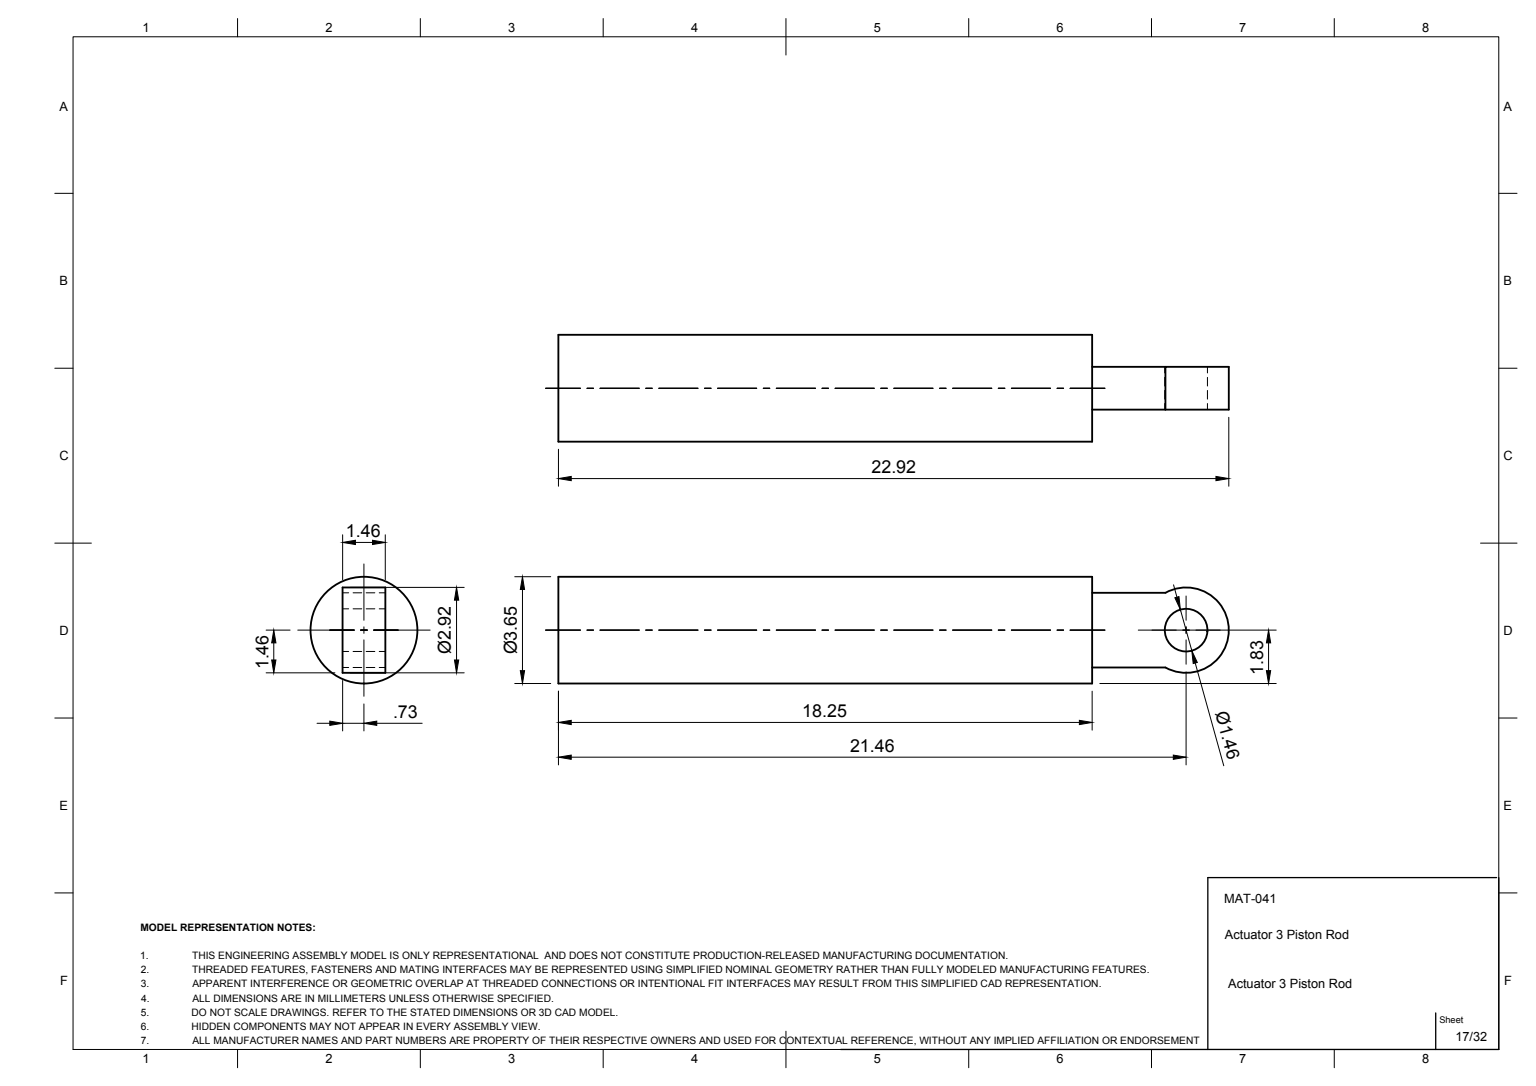
ISO-10303-21;
HEADER;
/* Generated by software containing ST-Developer
 * from STEP Tools, Inc. (www.steptools.com) 
 */

FILE_DESCRIPTION(
/* description */ ('STEP AP214'),
/* implementation_level */ '2;1');

FILE_NAME(
/* name */ 'Actuator 3 Piston Rod.step',
/* time_stamp */ '2026-11-14T21:57:47-08:00',
/* author */ (''),
/* organization */ (''),
/* preprocessor_version */ 'ST-DEVELOPER v20.2',
/* originating_system */ 'Autodesk Translation Framework v15.17.0.0',
/* authorisation */ '');

FILE_SCHEMA (('AUTOMOTIVE_DESIGN { 1 0 10303 214 3 1 1 }'));
ENDSEC;

DATA;
#10=MECHANICAL_DESIGN_GEOMETRIC_PRESENTATION_REPRESENTATION('',(#255),#13199);
#219=SHAPE_REPRESENTATION_RELATIONSHIP('SRR','None',#13289,#237);
#237=ADVANCED_BREP_SHAPE_REPRESENTATION('',(#273),#13185);
#255=STYLED_ITEM('',(#13411),#273);
#273=MANIFOLD_SOLID_BREP('Body1',#6850);
#335=FACE_BOUND('',#2475,.T.);
#336=FACE_BOUND('',#2478,.T.);
#337=FACE_BOUND('',#2481,.T.);
#505=PLANE('',#7523);
#506=PLANE('',#7524);
#507=PLANE('',#7525);
#508=PLANE('',#7526);
#509=PLANE('',#7527);
#510=PLANE('',#7528);
#898=LINE('',#11729,#1416);
#899=LINE('',#11736,#1417);
#900=LINE('',#11739,#1418);
#901=LINE('',#11744,#1419);
#902=LINE('',#11749,#1420);
#903=LINE('',#11751,#1421);
#904=LINE('',#11753,#1422);
#905=LINE('',#11754,#1423);
#906=LINE('',#11757,#1424);
#907=LINE('',#11758,#1425);
#908=LINE('',#11760,#1426);
#909=LINE('',#11762,#1427);
#1416=VECTOR('',#9029,0.730000000000001);
#1417=VECTOR('',#9036,1000.);
#1418=VECTOR('',#9039,1000.);
#1419=VECTOR('',#9044,1.825);
#1420=VECTOR('',#9049,1000.);
#1421=VECTOR('',#9050,1000.);
#1422=VECTOR('',#9051,1000.);
#1423=VECTOR('',#9052,1000.);
#1424=VECTOR('',#9057,1000.);
#1425=VECTOR('',#9058,1000.);
#1426=VECTOR('',#9061,1000.);
#1427=VECTOR('',#9064,1000.);
#1741=CYLINDRICAL_SURFACE('',#7514,0.730000000000001);
#1742=CYLINDRICAL_SURFACE('',#7517,1.46);
#1743=CYLINDRICAL_SURFACE('',#7520,1.825);
#2029=FACE_OUTER_BOUND('',#2471,.T.);
#2030=FACE_OUTER_BOUND('',#2472,.T.);
#2031=FACE_OUTER_BOUND('',#2473,.T.);
#2032=FACE_OUTER_BOUND('',#2474,.T.);
#2033=FACE_OUTER_BOUND('',#2476,.T.);
#2034=FACE_OUTER_BOUND('',#2477,.T.);
#2035=FACE_OUTER_BOUND('',#2479,.T.);
#2036=FACE_OUTER_BOUND('',#2480,.T.);
#2037=FACE_OUTER_BOUND('',#2482,.T.);
#2471=EDGE_LOOP('',(#5670,#5671,#5672,#5673));
#2472=EDGE_LOOP('',(#5674,#5675,#5676,#5677));
#2473=EDGE_LOOP('',(#5678,#5679,#5680,#5681));
#2474=EDGE_LOOP('',(#5682));
#2475=EDGE_LOOP('',(#5683,#5684,#5685,#5686));
#2476=EDGE_LOOP('',(#5687));
#2477=EDGE_LOOP('',(#5688,#5689,#5690,#5691));
#2478=EDGE_LOOP('',(#5692));
#2479=EDGE_LOOP('',(#5693,#5694,#5695,#5696));
#2480=EDGE_LOOP('',(#5697,#5698,#5699,#5700));
#2481=EDGE_LOOP('',(#5701));
#2482=EDGE_LOOP('',(#5702,#5703,#5704,#5705));
#2883=CIRCLE('',#7515,0.730000000000001);
#2884=CIRCLE('',#7516,0.730000000000001);
#2885=CIRCLE('',#7518,1.46);
#2886=CIRCLE('',#7519,1.46);
#2887=CIRCLE('',#7521,1.825);
#2888=CIRCLE('',#7522,1.825);
#3358=VERTEX_POINT('',#11726);
#3359=VERTEX_POINT('',#11728);
#3360=VERTEX_POINT('',#11732);
#3361=VERTEX_POINT('',#11733);
#3362=VERTEX_POINT('',#11735);
#3363=VERTEX_POINT('',#11737);
#3364=VERTEX_POINT('',#11741);
#3365=VERTEX_POINT('',#11743);
#3366=VERTEX_POINT('',#11747);
#3367=VERTEX_POINT('',#11748);
#3368=VERTEX_POINT('',#11750);
#3369=VERTEX_POINT('',#11752);
#4172=EDGE_CURVE('',#3358,#3358,#2883,.T.);
#4173=EDGE_CURVE('',#3358,#3359,#898,.T.);
#4174=EDGE_CURVE('',#3359,#3359,#2884,.T.);
#4175=EDGE_CURVE('',#3360,#3361,#2885,.T.);
#4176=EDGE_CURVE('',#3362,#3360,#899,.T.);
#4177=EDGE_CURVE('',#3363,#3362,#2886,.T.);
#4178=EDGE_CURVE('',#3361,#3363,#900,.T.);
#4179=EDGE_CURVE('',#3364,#3364,#2887,.T.);
#4180=EDGE_CURVE('',#3364,#3365,#901,.T.);
#4181=EDGE_CURVE('',#3365,#3365,#2888,.T.);
#4182=EDGE_CURVE('',#3366,#3367,#902,.T.);
#4183=EDGE_CURVE('',#3368,#3366,#903,.T.);
#4184=EDGE_CURVE('',#3369,#3368,#904,.T.);
#4185=EDGE_CURVE('',#3367,#3369,#905,.T.);
#4186=EDGE_CURVE('',#3363,#3366,#906,.T.);
#4187=EDGE_CURVE('',#3362,#3368,#907,.T.);
#4188=EDGE_CURVE('',#3361,#3367,#908,.T.);
#4189=EDGE_CURVE('',#3360,#3369,#909,.T.);
#5670=ORIENTED_EDGE('',*,*,#4172,.F.);
#5671=ORIENTED_EDGE('',*,*,#4173,.T.);
#5672=ORIENTED_EDGE('',*,*,#4174,.T.);
#5673=ORIENTED_EDGE('',*,*,#4173,.F.);
#5674=ORIENTED_EDGE('',*,*,#4175,.F.);
#5675=ORIENTED_EDGE('',*,*,#4176,.F.);
#5676=ORIENTED_EDGE('',*,*,#4177,.F.);
#5677=ORIENTED_EDGE('',*,*,#4178,.F.);
#5678=ORIENTED_EDGE('',*,*,#4179,.T.);
#5679=ORIENTED_EDGE('',*,*,#4180,.T.);
#5680=ORIENTED_EDGE('',*,*,#4181,.F.);
#5681=ORIENTED_EDGE('',*,*,#4180,.F.);
#5682=ORIENTED_EDGE('',*,*,#4181,.T.);
#5683=ORIENTED_EDGE('',*,*,#4182,.F.);
#5684=ORIENTED_EDGE('',*,*,#4183,.F.);
#5685=ORIENTED_EDGE('',*,*,#4184,.F.);
#5686=ORIENTED_EDGE('',*,*,#4185,.F.);
#5687=ORIENTED_EDGE('',*,*,#4179,.F.);
#5688=ORIENTED_EDGE('',*,*,#4186,.F.);
#5689=ORIENTED_EDGE('',*,*,#4177,.T.);
#5690=ORIENTED_EDGE('',*,*,#4187,.T.);
#5691=ORIENTED_EDGE('',*,*,#4183,.T.);
#5692=ORIENTED_EDGE('',*,*,#4174,.F.);
#5693=ORIENTED_EDGE('',*,*,#4188,.F.);
#5694=ORIENTED_EDGE('',*,*,#4178,.T.);
#5695=ORIENTED_EDGE('',*,*,#4186,.T.);
#5696=ORIENTED_EDGE('',*,*,#4182,.T.);
#5697=ORIENTED_EDGE('',*,*,#4175,.T.);
#5698=ORIENTED_EDGE('',*,*,#4188,.T.);
#5699=ORIENTED_EDGE('',*,*,#4185,.T.);
#5700=ORIENTED_EDGE('',*,*,#4189,.F.);
#5701=ORIENTED_EDGE('',*,*,#4172,.T.);
#5702=ORIENTED_EDGE('',*,*,#4187,.F.);
#5703=ORIENTED_EDGE('',*,*,#4176,.T.);
#5704=ORIENTED_EDGE('',*,*,#4189,.T.);
#5705=ORIENTED_EDGE('',*,*,#4184,.T.);
#6681=ADVANCED_FACE('',(#2029),#1741,.F.);
#6682=ADVANCED_FACE('',(#2030),#1742,.T.);
#6683=ADVANCED_FACE('',(#2031),#1743,.T.);
#6684=ADVANCED_FACE('',(#2032,#335),#505,.T.);
#6685=ADVANCED_FACE('',(#2033),#506,.F.);
#6686=ADVANCED_FACE('',(#2034,#336),#507,.F.);
#6687=ADVANCED_FACE('',(#2035),#508,.F.);
#6688=ADVANCED_FACE('',(#2036,#337),#509,.F.);
#6689=ADVANCED_FACE('',(#2037),#510,.F.);
#6850=CLOSED_SHELL('',(#6681,#6682,#6683,#6684,#6685,#6686,#6687,#6688,
#6689));
#7513=AXIS2_PLACEMENT_3D('',#11724,#9023,#9024);
#7514=AXIS2_PLACEMENT_3D('',#11725,#9025,#9026);
#7515=AXIS2_PLACEMENT_3D('',#11727,#9027,#9028);
#7516=AXIS2_PLACEMENT_3D('',#11730,#9030,#9031);
#7517=AXIS2_PLACEMENT_3D('',#11731,#9032,#9033);
#7518=AXIS2_PLACEMENT_3D('',#11734,#9034,#9035);
#7519=AXIS2_PLACEMENT_3D('',#11738,#9037,#9038);
#7520=AXIS2_PLACEMENT_3D('',#11740,#9040,#9041);
#7521=AXIS2_PLACEMENT_3D('',#11742,#9042,#9043);
#7522=AXIS2_PLACEMENT_3D('',#11745,#9045,#9046);
#7523=AXIS2_PLACEMENT_3D('',#11746,#9047,#9048);
#7524=AXIS2_PLACEMENT_3D('',#11755,#9053,#9054);
#7525=AXIS2_PLACEMENT_3D('',#11756,#9055,#9056);
#7526=AXIS2_PLACEMENT_3D('',#11759,#9059,#9060);
#7527=AXIS2_PLACEMENT_3D('',#11761,#9062,#9063);
#7528=AXIS2_PLACEMENT_3D('',#11763,#9065,#9066);
#9023=DIRECTION('axis',(0.,0.,1.));
#9024=DIRECTION('refdir',(1.,0.,0.));
#9025=DIRECTION('center_axis',(1.,1.23908819712629E-16,0.));
#9026=DIRECTION('ref_axis',(-1.23908819712629E-16,1.,0.));
#9027=DIRECTION('center_axis',(1.,1.23908819712629E-16,0.));
#9028=DIRECTION('ref_axis',(-1.23908819712629E-16,1.,0.));
#9029=DIRECTION('',(1.,1.23908819712629E-16,0.));
#9030=DIRECTION('center_axis',(1.,1.23908819712629E-16,0.));
#9031=DIRECTION('ref_axis',(-1.23908819712629E-16,1.,0.));
#9032=DIRECTION('center_axis',(1.,1.23908819712629E-16,0.));
#9033=DIRECTION('ref_axis',(-2.11060815823259E-32,6.12323399573677E-17,
1.));
#9034=DIRECTION('center_axis',(-1.,-1.23908819712629E-16,0.));
#9035=DIRECTION('ref_axis',(-1.23908819712629E-16,1.,0.));
#9036=DIRECTION('',(-1.,-1.23908819712629E-16,0.));
#9037=DIRECTION('center_axis',(1.,1.23908819712629E-16,0.));
#9038=DIRECTION('ref_axis',(-1.23908819712629E-16,1.,0.));
#9039=DIRECTION('',(1.,1.23908819712629E-16,0.));
#9040=DIRECTION('center_axis',(0.,0.,-1.));
#9041=DIRECTION('ref_axis',(-1.,0.,0.));
#9042=DIRECTION('center_axis',(0.,0.,1.));
#9043=DIRECTION('ref_axis',(1.,0.,0.));
#9044=DIRECTION('',(0.,0.,1.));
#9045=DIRECTION('center_axis',(0.,0.,1.));
#9046=DIRECTION('ref_axis',(1.,0.,0.));
#9047=DIRECTION('center_axis',(0.,0.,1.));
#9048=DIRECTION('ref_axis',(1.,0.,0.));
#9049=DIRECTION('',(-1.,0.,0.));
#9050=DIRECTION('',(-1.23908819712629E-16,1.,0.));
#9051=DIRECTION('',(1.,0.,0.));
#9052=DIRECTION('',(1.23908819712629E-16,-1.,0.));
#9053=DIRECTION('center_axis',(0.,0.,1.));
#9054=DIRECTION('ref_axis',(1.,0.,0.));
#9055=DIRECTION('center_axis',(-1.,-1.23908819712629E-16,0.));
#9056=DIRECTION('ref_axis',(1.23908819712629E-16,-1.,0.));
#9057=DIRECTION('',(0.,0.,-1.));
#9058=DIRECTION('',(0.,0.,-1.));
#9059=DIRECTION('center_axis',(0.,-1.,0.));
#9060=DIRECTION('ref_axis',(0.,0.,-1.));
#9061=DIRECTION('',(0.,0.,-1.));
#9062=DIRECTION('center_axis',(1.,1.23908819712629E-16,0.));
#9063=DIRECTION('ref_axis',(-1.23908819712629E-16,1.,0.));
#9064=DIRECTION('',(0.,0.,-1.));
#9065=DIRECTION('center_axis',(0.,1.,0.));
#9066=DIRECTION('ref_axis',(0.,0.,1.));
#11724=CARTESIAN_POINT('',(0.,0.,0.));
#11725=CARTESIAN_POINT('Origin',(-0.73,-5.37449520079003E-16,21.462));
#11726=CARTESIAN_POINT('',(-0.73,-0.730000000000002,21.462));
#11727=CARTESIAN_POINT('Origin',(-0.73,-5.37449520079003E-16,21.462));
#11728=CARTESIAN_POINT('',(0.73,-0.730000000000002,21.462));
#11729=CARTESIAN_POINT('',(-0.73,-0.730000000000002,21.462));
#11730=CARTESIAN_POINT('Origin',(0.73,-3.56542643298565E-16,21.462));
#11731=CARTESIAN_POINT('Origin',(-4.85950360212944,-1.04913143741791E-15,
21.462));
#11732=CARTESIAN_POINT('',(-0.73,-1.2775,20.7551805393172));
#11733=CARTESIAN_POINT('',(-0.73,1.2775,20.7551805393172));
#11734=CARTESIAN_POINT('Origin',(-0.73,-5.37449520079003E-16,21.462));
#11735=CARTESIAN_POINT('',(0.73,-1.2775,20.7551805393172));
#11736=CARTESIAN_POINT('',(-4.85950360212944,-1.2775,20.7551805393172));
#11737=CARTESIAN_POINT('',(0.73,1.2775,20.7551805393172));
#11738=CARTESIAN_POINT('Origin',(0.73,-3.56542643298565E-16,21.462));
#11739=CARTESIAN_POINT('',(-4.85950360212944,1.2775,20.7551805393172));
#11740=CARTESIAN_POINT('Origin',(0.,0.,18.25));
#11741=CARTESIAN_POINT('',(1.825,-2.23498040844392E-16,-2.22044604925031E-15));
#11742=CARTESIAN_POINT('Origin',(0.,0.,0.));
#11743=CARTESIAN_POINT('',(1.825,-2.23498040844392E-16,18.25));
#11744=CARTESIAN_POINT('',(1.825,-2.23498040844392E-16,18.25));
#11745=CARTESIAN_POINT('Origin',(0.,0.,18.25));
#11746=CARTESIAN_POINT('Origin',(0.,0.,18.25));
#11747=CARTESIAN_POINT('',(0.73,1.2775,18.25));
#11748=CARTESIAN_POINT('',(-0.73,1.2775,18.25));
#11749=CARTESIAN_POINT('',(-0.73,1.2775,18.25));
#11750=CARTESIAN_POINT('',(0.73,-1.2775,18.25));
#11751=CARTESIAN_POINT('',(0.73,1.2775,18.25));
#11752=CARTESIAN_POINT('',(-0.73,-1.2775,18.25));
#11753=CARTESIAN_POINT('',(-0.73,-1.2775,18.25));
#11754=CARTESIAN_POINT('',(-0.73,1.2775,18.25));
#11755=CARTESIAN_POINT('Origin',(0.,0.,0.));
#11756=CARTESIAN_POINT('Origin',(0.73,1.2775,21.462));
#11757=CARTESIAN_POINT('',(0.73,1.2775,21.462));
#11758=CARTESIAN_POINT('',(0.73,-1.2775,21.462));
#11759=CARTESIAN_POINT('Origin',(-0.73,1.2775,21.462));
#11760=CARTESIAN_POINT('',(-0.73,1.2775,21.462));
#11761=CARTESIAN_POINT('Origin',(-0.73,1.2775,21.462));
#11762=CARTESIAN_POINT('',(-0.73,-1.2775,21.462));
#11763=CARTESIAN_POINT('Origin',(-0.73,-1.2775,21.462));
#13159=UNCERTAINTY_MEASURE_WITH_UNIT(LENGTH_MEASURE(0.01),#13200,
'DISTANCE_ACCURACY_VALUE',
'Maximum model space distance between geometric entities at asserted c
onnectivities');
#13173=UNCERTAINTY_MEASURE_WITH_UNIT(LENGTH_MEASURE(0.01),#13200,
'DISTANCE_ACCURACY_VALUE',
'Maximum model space distance between geometric entities at asserted c
onnectivities');
#13185=(
GEOMETRIC_REPRESENTATION_CONTEXT(3)
GLOBAL_UNCERTAINTY_ASSIGNED_CONTEXT((#13159))
GLOBAL_UNIT_ASSIGNED_CONTEXT((#13200,#13202,#13203))
REPRESENTATION_CONTEXT('','3D')
);
#13199=(
GEOMETRIC_REPRESENTATION_CONTEXT(3)
GLOBAL_UNCERTAINTY_ASSIGNED_CONTEXT((#13173))
GLOBAL_UNIT_ASSIGNED_CONTEXT((#13200,#13202,#13203))
REPRESENTATION_CONTEXT('','3D')
);
#13200=(
LENGTH_UNIT()
NAMED_UNIT(*)
SI_UNIT(.MILLI.,.METRE.)
);
#13202=(
NAMED_UNIT(*)
PLANE_ANGLE_UNIT()
SI_UNIT($,.RADIAN.)
);
#13203=(
NAMED_UNIT(*)
SI_UNIT($,.STERADIAN.)
SOLID_ANGLE_UNIT()
);
#13215=SHAPE_DEFINITION_REPRESENTATION(#13242,#13289);
#13242=PRODUCT_DEFINITION_SHAPE('',$,#13315);
#13289=SHAPE_REPRESENTATION('',(#7513),#13185);
#13303=PRODUCT_DEFINITION_CONTEXT('part definition',#13380,'design');
#13315=PRODUCT_DEFINITION('Actuator 3 Piston Rod',
'Actuator 3 Piston Rod',#13340,#13303);
#13340=PRODUCT_DEFINITION_FORMATION('',$,#13393);
#13380=APPLICATION_CONTEXT(
'Core Data for Automotive Mechanical Design Process');
#13381=PRODUCT_CONTEXT('part definition',#13380,'mechanical');
#13393=PRODUCT('Actuator 3 Piston Rod','Actuator 3 Piston Rod',$,(#13381));
#13411=PRESENTATION_STYLE_ASSIGNMENT((#13416));
#13416=SURFACE_STYLE_USAGE(.BOTH.,#13421);
#13421=SURFACE_SIDE_STYLE('',(#13426));
#13426=SURFACE_STYLE_FILL_AREA(#13431);
#13431=FILL_AREA_STYLE('Opaque(97,158,199)',(#13436));
#13436=FILL_AREA_STYLE_COLOUR('Opaque(97,158,199)',#13441);
#13441=COLOUR_RGB('Opaque(97,158,199)',0.380392156862745,0.619607843137255,
0.780392156862745);
ENDSEC;
END-ISO-10303-21;
